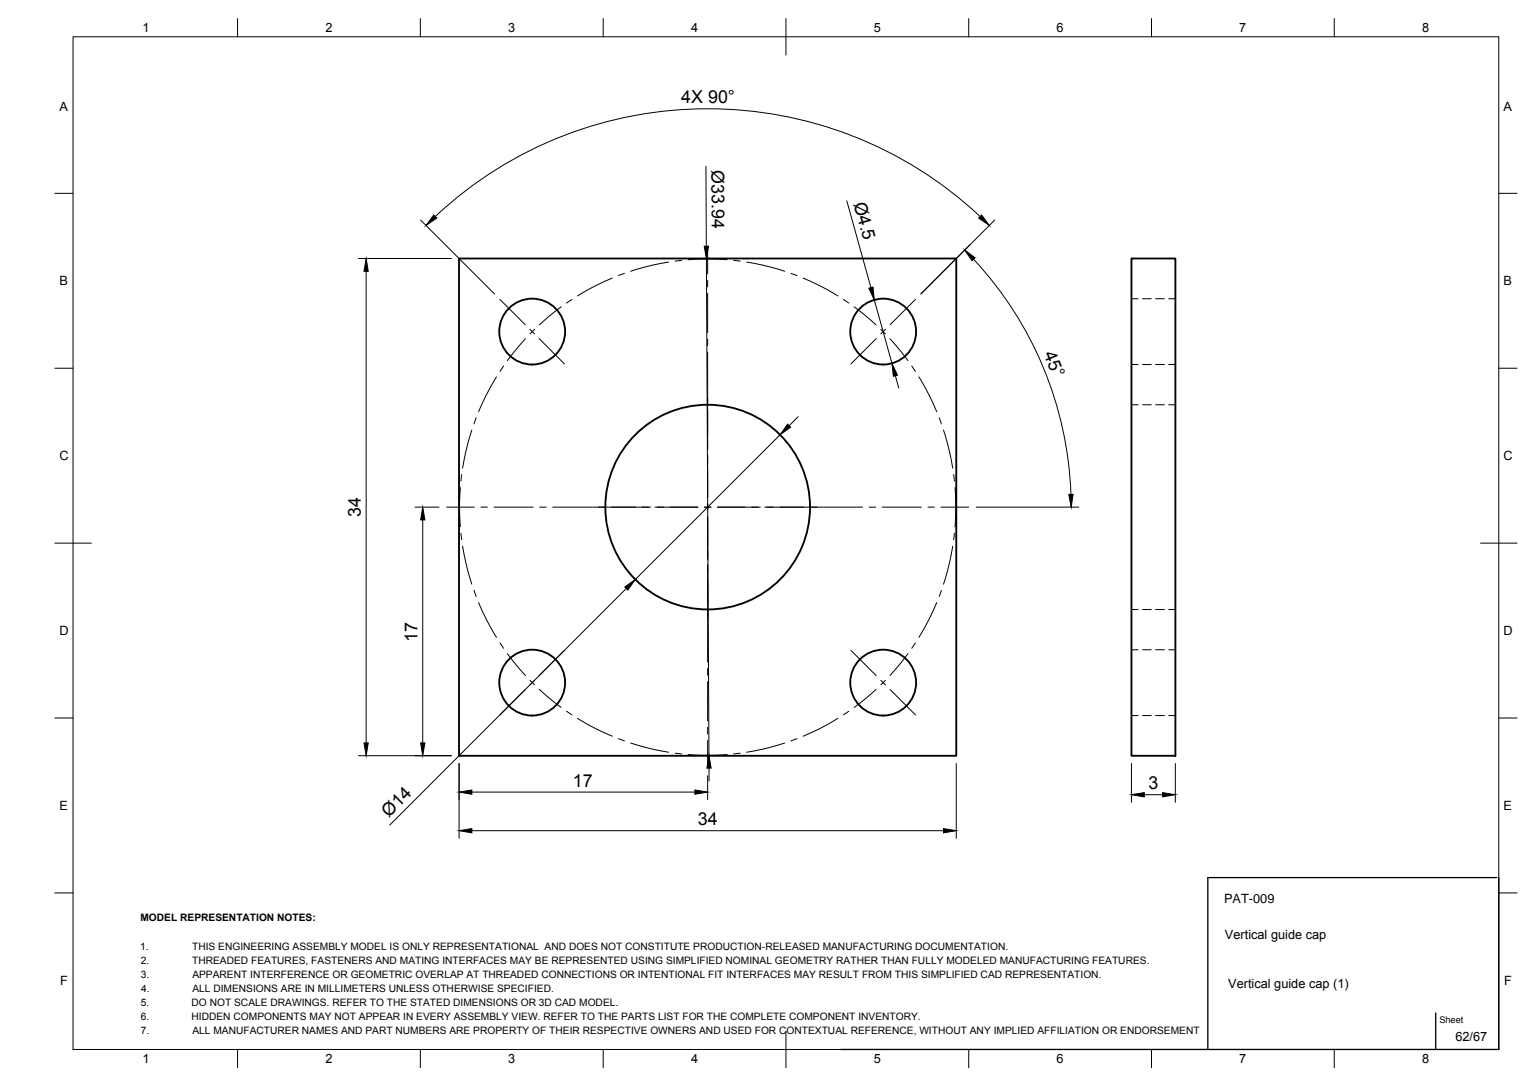
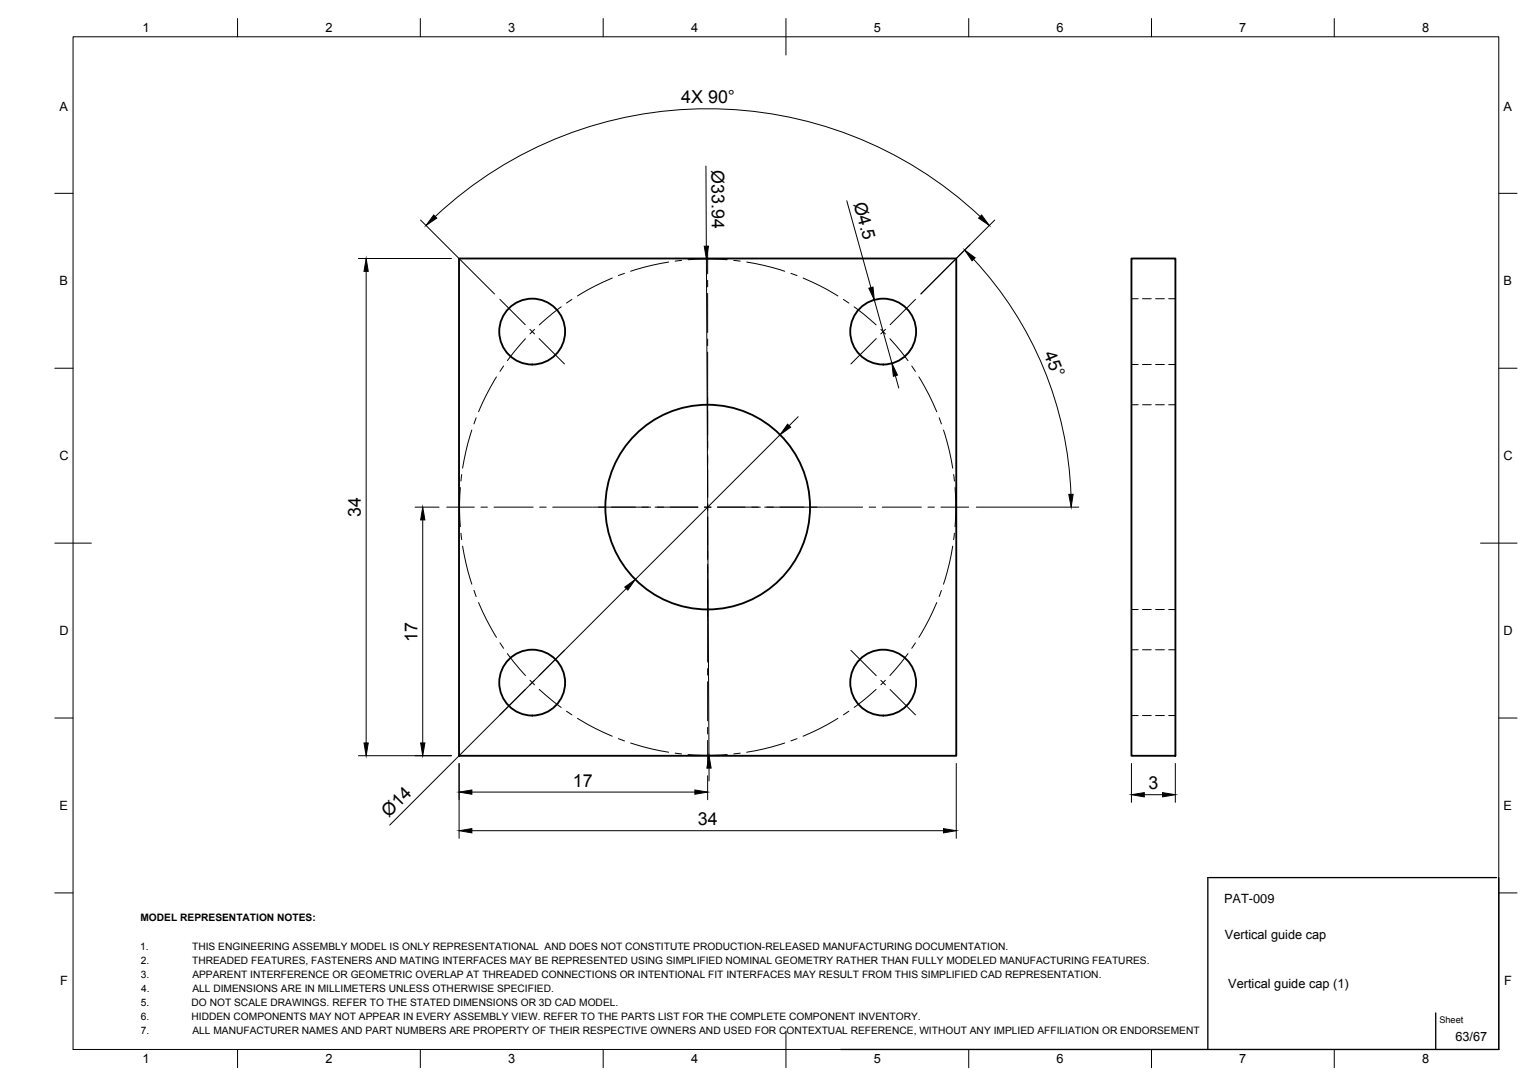
ISO-10303-21;
HEADER;
/* Generated by software containing ST-Developer
 * from STEP Tools, Inc. (www.steptools.com) 
 */

FILE_DESCRIPTION(
/* description */ ('Bell-crank linkage with push rods'),
/* implementation_level */ '2;1');

FILE_NAME(
/* name */ 'Vertical guide cap.step',
/* time_stamp */ '2026-10-28T03:25:15-07:00',
/* author */ (''),
/* organization */ (''),
/* preprocessor_version */ 'ST-DEVELOPER v20.2',
/* originating_system */ 'Autodesk Translation Framework v15.17.0.0',
/* authorisation */ '');

FILE_SCHEMA (('AUTOMOTIVE_DESIGN { 1 0 10303 214 3 1 1 }'));
ENDSEC;

DATA;
#10=MECHANICAL_DESIGN_GEOMETRIC_PRESENTATION_REPRESENTATION('',(#657),#16678);
#541=SHAPE_REPRESENTATION_RELATIONSHIP('SRR','None',#16963,#595);
#595=ADVANCED_BREP_SHAPE_REPRESENTATION('',(#717),#16668);
#657=STYLED_ITEM('',(#17277),#717);
#717=MANIFOLD_SOLID_BREP('Body1',#8849);
#925=FACE_BOUND('',#2413,.T.);
#926=FACE_BOUND('',#2414,.T.);
#927=FACE_BOUND('',#2415,.T.);
#928=FACE_BOUND('',#2416,.T.);
#929=FACE_BOUND('',#2417,.T.);
#930=FACE_BOUND('',#2420,.T.);
#931=FACE_BOUND('',#2421,.T.);
#932=FACE_BOUND('',#2422,.T.);
#933=FACE_BOUND('',#2423,.T.);
#934=FACE_BOUND('',#2424,.T.);
#1196=PLANE('',#10393);
#1197=PLANE('',#10394);
#1198=PLANE('',#10395);
#1199=PLANE('',#10396);
#1200=PLANE('',#10397);
#1201=PLANE('',#10398);
#1685=FACE_OUTER_BOUND('',#2407,.T.);
#1686=FACE_OUTER_BOUND('',#2408,.T.);
#1687=FACE_OUTER_BOUND('',#2409,.T.);
#1688=FACE_OUTER_BOUND('',#2410,.T.);
#1689=FACE_OUTER_BOUND('',#2411,.T.);
#1690=FACE_OUTER_BOUND('',#2412,.T.);
#1691=FACE_OUTER_BOUND('',#2418,.T.);
#1692=FACE_OUTER_BOUND('',#2419,.T.);
#1693=FACE_OUTER_BOUND('',#2425,.T.);
#1694=FACE_OUTER_BOUND('',#2426,.T.);
#1695=FACE_OUTER_BOUND('',#2427,.T.);
#2407=EDGE_LOOP('',(#7743,#7744,#7745,#7746));
#2408=EDGE_LOOP('',(#7747,#7748,#7749,#7750));
#2409=EDGE_LOOP('',(#7751,#7752,#7753,#7754));
#2410=EDGE_LOOP('',(#7755,#7756,#7757,#7758));
#2411=EDGE_LOOP('',(#7759,#7760,#7761,#7762));
#2412=EDGE_LOOP('',(#7763,#7764,#7765,#7766));
#2413=EDGE_LOOP('',(#7767));
#2414=EDGE_LOOP('',(#7768));
#2415=EDGE_LOOP('',(#7769));
#2416=EDGE_LOOP('',(#7770));
#2417=EDGE_LOOP('',(#7771));
#2418=EDGE_LOOP('',(#7772,#7773,#7774,#7775));
#2419=EDGE_LOOP('',(#7776,#7777,#7778,#7779));
#2420=EDGE_LOOP('',(#7780));
#2421=EDGE_LOOP('',(#7781));
#2422=EDGE_LOOP('',(#7782));
#2423=EDGE_LOOP('',(#7783));
#2424=EDGE_LOOP('',(#7784));
#2425=EDGE_LOOP('',(#7785,#7786,#7787,#7788));
#2426=EDGE_LOOP('',(#7789,#7790,#7791,#7792));
#2427=EDGE_LOOP('',(#7793,#7794,#7795,#7796));
#2988=LINE('',#16103,#3537);
#2989=LINE('',#16109,#3538);
#2990=LINE('',#16115,#3539);
#2991=LINE('',#16121,#3540);
#2992=LINE('',#16127,#3541);
#2993=LINE('',#16132,#3542);
#2994=LINE('',#16134,#3543);
#2995=LINE('',#16136,#3544);
#2996=LINE('',#16137,#3545);
#2997=LINE('',#16140,#3546);
#2998=LINE('',#16142,#3547);
#2999=LINE('',#16143,#3548);
#3000=LINE('',#16146,#3549);
#3001=LINE('',#16148,#3550);
#3002=LINE('',#16149,#3551);
#3003=LINE('',#16151,#3552);
#3004=LINE('',#16152,#3553);
#3537=VECTOR('',#12938,0.225);
#3538=VECTOR('',#12945,0.225);
#3539=VECTOR('',#12952,0.225);
#3540=VECTOR('',#12959,0.225);
#3541=VECTOR('',#12966,0.7);
#3542=VECTOR('',#12971,1.);
#3543=VECTOR('',#12972,1.);
#3544=VECTOR('',#12973,1.);
#3545=VECTOR('',#12974,1.);
#3546=VECTOR('',#12977,1.);
#3547=VECTOR('',#12978,1.);
#3548=VECTOR('',#12979,1.);
#3549=VECTOR('',#12982,1.);
#3550=VECTOR('',#12983,1.);
#3551=VECTOR('',#12984,1.);
#3552=VECTOR('',#12987,1.);
#3553=VECTOR('',#12988,1.);
#4051=CIRCLE('',#10379,0.225);
#4052=CIRCLE('',#10380,0.225);
#4053=CIRCLE('',#10382,0.225);
#4054=CIRCLE('',#10383,0.225);
#4055=CIRCLE('',#10385,0.225);
#4056=CIRCLE('',#10386,0.225);
#4057=CIRCLE('',#10388,0.225);
#4058=CIRCLE('',#10389,0.225);
#4059=CIRCLE('',#10391,0.7);
#4060=CIRCLE('',#10392,0.7);
#4726=VERTEX_POINT('',#16100);
#4727=VERTEX_POINT('',#16102);
#4728=VERTEX_POINT('',#16106);
#4729=VERTEX_POINT('',#16108);
#4730=VERTEX_POINT('',#16112);
#4731=VERTEX_POINT('',#16114);
#4732=VERTEX_POINT('',#16118);
#4733=VERTEX_POINT('',#16120);
#4734=VERTEX_POINT('',#16124);
#4735=VERTEX_POINT('',#16126);
#4736=VERTEX_POINT('',#16130);
#4737=VERTEX_POINT('',#16131);
#4738=VERTEX_POINT('',#16133);
#4739=VERTEX_POINT('',#16135);
#4740=VERTEX_POINT('',#16139);
#4741=VERTEX_POINT('',#16141);
#4742=VERTEX_POINT('',#16145);
#4743=VERTEX_POINT('',#16147);
#5749=EDGE_CURVE('',#4726,#4726,#4051,.T.);
#5750=EDGE_CURVE('',#4726,#4727,#2988,.T.);
#5751=EDGE_CURVE('',#4727,#4727,#4052,.T.);
#5752=EDGE_CURVE('',#4728,#4728,#4053,.T.);
#5753=EDGE_CURVE('',#4728,#4729,#2989,.T.);
#5754=EDGE_CURVE('',#4729,#4729,#4054,.T.);
#5755=EDGE_CURVE('',#4730,#4730,#4055,.T.);
#5756=EDGE_CURVE('',#4730,#4731,#2990,.T.);
#5757=EDGE_CURVE('',#4731,#4731,#4056,.T.);
#5758=EDGE_CURVE('',#4732,#4732,#4057,.T.);
#5759=EDGE_CURVE('',#4732,#4733,#2991,.T.);
#5760=EDGE_CURVE('',#4733,#4733,#4058,.T.);
#5761=EDGE_CURVE('',#4734,#4734,#4059,.T.);
#5762=EDGE_CURVE('',#4734,#4735,#2992,.T.);
#5763=EDGE_CURVE('',#4735,#4735,#4060,.T.);
#5764=EDGE_CURVE('',#4736,#4737,#2993,.T.);
#5765=EDGE_CURVE('',#4737,#4738,#2994,.T.);
#5766=EDGE_CURVE('',#4739,#4738,#2995,.T.);
#5767=EDGE_CURVE('',#4736,#4739,#2996,.T.);
#5768=EDGE_CURVE('',#4740,#4736,#2997,.T.);
#5769=EDGE_CURVE('',#4741,#4739,#2998,.T.);
#5770=EDGE_CURVE('',#4740,#4741,#2999,.T.);
#5771=EDGE_CURVE('',#4742,#4740,#3000,.T.);
#5772=EDGE_CURVE('',#4743,#4741,#3001,.T.);
#5773=EDGE_CURVE('',#4742,#4743,#3002,.T.);
#5774=EDGE_CURVE('',#4737,#4742,#3003,.T.);
#5775=EDGE_CURVE('',#4738,#4743,#3004,.T.);
#7743=ORIENTED_EDGE('',*,*,#5749,.F.);
#7744=ORIENTED_EDGE('',*,*,#5750,.T.);
#7745=ORIENTED_EDGE('',*,*,#5751,.F.);
#7746=ORIENTED_EDGE('',*,*,#5750,.F.);
#7747=ORIENTED_EDGE('',*,*,#5752,.F.);
#7748=ORIENTED_EDGE('',*,*,#5753,.T.);
#7749=ORIENTED_EDGE('',*,*,#5754,.F.);
#7750=ORIENTED_EDGE('',*,*,#5753,.F.);
#7751=ORIENTED_EDGE('',*,*,#5755,.F.);
#7752=ORIENTED_EDGE('',*,*,#5756,.T.);
#7753=ORIENTED_EDGE('',*,*,#5757,.F.);
#7754=ORIENTED_EDGE('',*,*,#5756,.F.);
#7755=ORIENTED_EDGE('',*,*,#5758,.F.);
#7756=ORIENTED_EDGE('',*,*,#5759,.T.);
#7757=ORIENTED_EDGE('',*,*,#5760,.F.);
#7758=ORIENTED_EDGE('',*,*,#5759,.F.);
#7759=ORIENTED_EDGE('',*,*,#5761,.F.);
#7760=ORIENTED_EDGE('',*,*,#5762,.T.);
#7761=ORIENTED_EDGE('',*,*,#5763,.F.);
#7762=ORIENTED_EDGE('',*,*,#5762,.F.);
#7763=ORIENTED_EDGE('',*,*,#5764,.T.);
#7764=ORIENTED_EDGE('',*,*,#5765,.T.);
#7765=ORIENTED_EDGE('',*,*,#5766,.F.);
#7766=ORIENTED_EDGE('',*,*,#5767,.F.);
#7767=ORIENTED_EDGE('',*,*,#5763,.T.);
#7768=ORIENTED_EDGE('',*,*,#5760,.T.);
#7769=ORIENTED_EDGE('',*,*,#5757,.T.);
#7770=ORIENTED_EDGE('',*,*,#5754,.T.);
#7771=ORIENTED_EDGE('',*,*,#5751,.T.);
#7772=ORIENTED_EDGE('',*,*,#5768,.T.);
#7773=ORIENTED_EDGE('',*,*,#5767,.T.);
#7774=ORIENTED_EDGE('',*,*,#5769,.F.);
#7775=ORIENTED_EDGE('',*,*,#5770,.F.);
#7776=ORIENTED_EDGE('',*,*,#5771,.T.);
#7777=ORIENTED_EDGE('',*,*,#5770,.T.);
#7778=ORIENTED_EDGE('',*,*,#5772,.F.);
#7779=ORIENTED_EDGE('',*,*,#5773,.F.);
#7780=ORIENTED_EDGE('',*,*,#5761,.T.);
#7781=ORIENTED_EDGE('',*,*,#5758,.T.);
#7782=ORIENTED_EDGE('',*,*,#5755,.T.);
#7783=ORIENTED_EDGE('',*,*,#5752,.T.);
#7784=ORIENTED_EDGE('',*,*,#5749,.T.);
#7785=ORIENTED_EDGE('',*,*,#5774,.T.);
#7786=ORIENTED_EDGE('',*,*,#5773,.T.);
#7787=ORIENTED_EDGE('',*,*,#5775,.F.);
#7788=ORIENTED_EDGE('',*,*,#5765,.F.);
#7789=ORIENTED_EDGE('',*,*,#5775,.T.);
#7790=ORIENTED_EDGE('',*,*,#5772,.T.);
#7791=ORIENTED_EDGE('',*,*,#5769,.T.);
#7792=ORIENTED_EDGE('',*,*,#5766,.T.);
#7793=ORIENTED_EDGE('',*,*,#5774,.F.);
#7794=ORIENTED_EDGE('',*,*,#5764,.F.);
#7795=ORIENTED_EDGE('',*,*,#5768,.F.);
#7796=ORIENTED_EDGE('',*,*,#5771,.F.);
#8242=CYLINDRICAL_SURFACE('',#10378,0.225);
#8243=CYLINDRICAL_SURFACE('',#10381,0.225);
#8244=CYLINDRICAL_SURFACE('',#10384,0.225);
#8245=CYLINDRICAL_SURFACE('',#10387,0.225);
#8246=CYLINDRICAL_SURFACE('',#10390,0.7);
#8710=ADVANCED_FACE('',(#1685),#8242,.F.);
#8711=ADVANCED_FACE('',(#1686),#8243,.F.);
#8712=ADVANCED_FACE('',(#1687),#8244,.F.);
#8713=ADVANCED_FACE('',(#1688),#8245,.F.);
#8714=ADVANCED_FACE('',(#1689),#8246,.F.);
#8715=ADVANCED_FACE('',(#1690,#925,#926,#927,#928,#929),#1196,.T.);
#8716=ADVANCED_FACE('',(#1691),#1197,.T.);
#8717=ADVANCED_FACE('',(#1692,#930,#931,#932,#933,#934),#1198,.T.);
#8718=ADVANCED_FACE('',(#1693),#1199,.T.);
#8719=ADVANCED_FACE('',(#1694),#1200,.T.);
#8720=ADVANCED_FACE('',(#1695),#1201,.F.);
#8849=CLOSED_SHELL('',(#8710,#8711,#8712,#8713,#8714,#8715,#8716,#8717,
#8718,#8719,#8720));
#10377=AXIS2_PLACEMENT_3D('',#16098,#12932,#12933);
#10378=AXIS2_PLACEMENT_3D('',#16099,#12934,#12935);
#10379=AXIS2_PLACEMENT_3D('',#16101,#12936,#12937);
#10380=AXIS2_PLACEMENT_3D('',#16104,#12939,#12940);
#10381=AXIS2_PLACEMENT_3D('',#16105,#12941,#12942);
#10382=AXIS2_PLACEMENT_3D('',#16107,#12943,#12944);
#10383=AXIS2_PLACEMENT_3D('',#16110,#12946,#12947);
#10384=AXIS2_PLACEMENT_3D('',#16111,#12948,#12949);
#10385=AXIS2_PLACEMENT_3D('',#16113,#12950,#12951);
#10386=AXIS2_PLACEMENT_3D('',#16116,#12953,#12954);
#10387=AXIS2_PLACEMENT_3D('',#16117,#12955,#12956);
#10388=AXIS2_PLACEMENT_3D('',#16119,#12957,#12958);
#10389=AXIS2_PLACEMENT_3D('',#16122,#12960,#12961);
#10390=AXIS2_PLACEMENT_3D('',#16123,#12962,#12963);
#10391=AXIS2_PLACEMENT_3D('',#16125,#12964,#12965);
#10392=AXIS2_PLACEMENT_3D('',#16128,#12967,#12968);
#10393=AXIS2_PLACEMENT_3D('',#16129,#12969,#12970);
#10394=AXIS2_PLACEMENT_3D('',#16138,#12975,#12976);
#10395=AXIS2_PLACEMENT_3D('',#16144,#12980,#12981);
#10396=AXIS2_PLACEMENT_3D('',#16150,#12985,#12986);
#10397=AXIS2_PLACEMENT_3D('',#16153,#12989,#12990);
#10398=AXIS2_PLACEMENT_3D('',#16154,#12991,#12992);
#12932=DIRECTION('axis',(0.,0.,1.));
#12933=DIRECTION('refdir',(1.,0.,0.));
#12934=DIRECTION('center_axis',(0.,1.,0.));
#12935=DIRECTION('ref_axis',(1.,0.,0.));
#12936=DIRECTION('center_axis',(0.,1.,0.));
#12937=DIRECTION('ref_axis',(1.,0.,0.));
#12938=DIRECTION('',(0.,1.,0.));
#12939=DIRECTION('center_axis',(0.,-1.,0.));
#12940=DIRECTION('ref_axis',(1.,0.,0.));
#12941=DIRECTION('center_axis',(0.,1.,0.));
#12942=DIRECTION('ref_axis',(1.,0.,0.));
#12943=DIRECTION('center_axis',(0.,1.,0.));
#12944=DIRECTION('ref_axis',(1.,0.,0.));
#12945=DIRECTION('',(0.,1.,0.));
#12946=DIRECTION('center_axis',(0.,-1.,0.));
#12947=DIRECTION('ref_axis',(1.,0.,0.));
#12948=DIRECTION('center_axis',(0.,1.,0.));
#12949=DIRECTION('ref_axis',(1.,0.,0.));
#12950=DIRECTION('center_axis',(0.,1.,0.));
#12951=DIRECTION('ref_axis',(1.,0.,0.));
#12952=DIRECTION('',(0.,1.,0.));
#12953=DIRECTION('center_axis',(0.,-1.,0.));
#12954=DIRECTION('ref_axis',(1.,0.,0.));
#12955=DIRECTION('center_axis',(0.,1.,0.));
#12956=DIRECTION('ref_axis',(1.,0.,0.));
#12957=DIRECTION('center_axis',(0.,1.,0.));
#12958=DIRECTION('ref_axis',(1.,0.,0.));
#12959=DIRECTION('',(0.,1.,0.));
#12960=DIRECTION('center_axis',(0.,-1.,0.));
#12961=DIRECTION('ref_axis',(1.,0.,0.));
#12962=DIRECTION('center_axis',(0.,1.,0.));
#12963=DIRECTION('ref_axis',(1.,0.,0.));
#12964=DIRECTION('center_axis',(0.,1.,0.));
#12965=DIRECTION('ref_axis',(1.,0.,0.));
#12966=DIRECTION('',(0.,1.,0.));
#12967=DIRECTION('center_axis',(0.,-1.,0.));
#12968=DIRECTION('ref_axis',(1.,0.,0.));
#12969=DIRECTION('center_axis',(0.,1.,0.));
#12970=DIRECTION('ref_axis',(-1.,0.,0.));
#12971=DIRECTION('',(-1.,0.,0.));
#12972=DIRECTION('',(0.,0.,1.));
#12973=DIRECTION('',(-1.,0.,0.));
#12974=DIRECTION('',(0.,0.,1.));
#12975=DIRECTION('center_axis',(1.,0.,0.));
#12976=DIRECTION('ref_axis',(0.,1.,0.));
#12977=DIRECTION('',(0.,1.,0.));
#12978=DIRECTION('',(0.,1.,0.));
#12979=DIRECTION('',(0.,0.,1.));
#12980=DIRECTION('center_axis',(0.,-1.,0.));
#12981=DIRECTION('ref_axis',(1.,0.,0.));
#12982=DIRECTION('',(1.,0.,0.));
#12983=DIRECTION('',(1.,0.,0.));
#12984=DIRECTION('',(0.,0.,1.));
#12985=DIRECTION('center_axis',(-1.,0.,0.));
#12986=DIRECTION('ref_axis',(0.,-1.,0.));
#12987=DIRECTION('',(0.,-1.,0.));
#12988=DIRECTION('',(0.,-1.,0.));
#12989=DIRECTION('center_axis',(0.,0.,1.));
#12990=DIRECTION('ref_axis',(1.,0.,0.));
#12991=DIRECTION('center_axis',(0.,0.,1.));
#12992=DIRECTION('ref_axis',(1.,0.,0.));
#16098=CARTESIAN_POINT('',(0.,0.,0.));
#16099=CARTESIAN_POINT('Origin',(5.2,10.1,2.8));
#16100=CARTESIAN_POINT('',(4.975,10.2,2.8));
#16101=CARTESIAN_POINT('Origin',(5.2,10.2,2.8));
#16102=CARTESIAN_POINT('',(4.975,10.5,2.8));
#16103=CARTESIAN_POINT('',(4.975,10.1,2.8));
#16104=CARTESIAN_POINT('Origin',(5.2,10.5,2.8));
#16105=CARTESIAN_POINT('Origin',(2.8,10.1,5.2));
#16106=CARTESIAN_POINT('',(2.575,10.2,5.2));
#16107=CARTESIAN_POINT('Origin',(2.8,10.2,5.2));
#16108=CARTESIAN_POINT('',(2.575,10.5,5.2));
#16109=CARTESIAN_POINT('',(2.575,10.1,5.2));
#16110=CARTESIAN_POINT('Origin',(2.8,10.5,5.2));
#16111=CARTESIAN_POINT('Origin',(2.8,10.1,2.8));
#16112=CARTESIAN_POINT('',(2.575,10.2,2.8));
#16113=CARTESIAN_POINT('Origin',(2.8,10.2,2.8));
#16114=CARTESIAN_POINT('',(2.575,10.5,2.8));
#16115=CARTESIAN_POINT('',(2.575,10.1,2.8));
#16116=CARTESIAN_POINT('Origin',(2.8,10.5,2.8));
#16117=CARTESIAN_POINT('Origin',(5.2,10.1,5.2));
#16118=CARTESIAN_POINT('',(4.975,10.2,5.2));
#16119=CARTESIAN_POINT('Origin',(5.2,10.2,5.2));
#16120=CARTESIAN_POINT('',(4.975,10.5,5.2));
#16121=CARTESIAN_POINT('',(4.975,10.1,5.2));
#16122=CARTESIAN_POINT('Origin',(5.2,10.5,5.2));
#16123=CARTESIAN_POINT('Origin',(4.,10.1,4.));
#16124=CARTESIAN_POINT('',(3.3,10.2,4.));
#16125=CARTESIAN_POINT('Origin',(4.,10.2,4.));
#16126=CARTESIAN_POINT('',(3.3,10.5,4.));
#16127=CARTESIAN_POINT('',(3.3,10.1,4.));
#16128=CARTESIAN_POINT('Origin',(4.,10.5,4.));
#16129=CARTESIAN_POINT('Origin',(5.7,10.5,2.3));
#16130=CARTESIAN_POINT('',(5.7,10.5,2.3));
#16131=CARTESIAN_POINT('',(2.3,10.5,2.3));
#16132=CARTESIAN_POINT('',(5.7,10.5,2.3));
#16133=CARTESIAN_POINT('',(2.3,10.5,5.7));
#16134=CARTESIAN_POINT('',(2.3,10.5,2.3));
#16135=CARTESIAN_POINT('',(5.7,10.5,5.7));
#16136=CARTESIAN_POINT('',(5.7,10.5,5.7));
#16137=CARTESIAN_POINT('',(5.7,10.5,2.3));
#16138=CARTESIAN_POINT('Origin',(5.7,10.2,2.3));
#16139=CARTESIAN_POINT('',(5.7,10.2,2.3));
#16140=CARTESIAN_POINT('',(5.7,10.2,2.3));
#16141=CARTESIAN_POINT('',(5.7,10.2,5.7));
#16142=CARTESIAN_POINT('',(5.7,10.2,5.7));
#16143=CARTESIAN_POINT('',(5.7,10.2,2.3));
#16144=CARTESIAN_POINT('Origin',(2.3,10.2,2.3));
#16145=CARTESIAN_POINT('',(2.3,10.2,2.3));
#16146=CARTESIAN_POINT('',(2.3,10.2,2.3));
#16147=CARTESIAN_POINT('',(2.3,10.2,5.7));
#16148=CARTESIAN_POINT('',(2.3,10.2,5.7));
#16149=CARTESIAN_POINT('',(2.3,10.2,2.3));
#16150=CARTESIAN_POINT('Origin',(2.3,10.5,2.3));
#16151=CARTESIAN_POINT('',(2.3,10.5,2.3));
#16152=CARTESIAN_POINT('',(2.3,10.5,5.7));
#16153=CARTESIAN_POINT('Origin',(4.,10.35,5.7));
#16154=CARTESIAN_POINT('Origin',(4.,10.35,2.3));
#16604=UNCERTAINTY_MEASURE_WITH_UNIT(LENGTH_MEASURE(0.001),#16679,
'DISTANCE_ACCURACY_VALUE',
'Maximum model space distance between geometric entities at asserted c
onnectivities');
#16614=UNCERTAINTY_MEASURE_WITH_UNIT(LENGTH_MEASURE(0.001),#16679,
'DISTANCE_ACCURACY_VALUE',
'Maximum model space distance between geometric entities at asserted c
onnectivities');
#16668=(
GEOMETRIC_REPRESENTATION_CONTEXT(3)
GLOBAL_UNCERTAINTY_ASSIGNED_CONTEXT((#16604))
GLOBAL_UNIT_ASSIGNED_CONTEXT((#16679,#16681,#16682))
REPRESENTATION_CONTEXT('','3D')
);
#16678=(
GEOMETRIC_REPRESENTATION_CONTEXT(3)
GLOBAL_UNCERTAINTY_ASSIGNED_CONTEXT((#16614))
GLOBAL_UNIT_ASSIGNED_CONTEXT((#16679,#16681,#16682))
REPRESENTATION_CONTEXT('','3D')
);
#16679=(
LENGTH_UNIT()
NAMED_UNIT(*)
SI_UNIT(.CENTI.,.METRE.)
);
#16681=(
NAMED_UNIT(*)
PLANE_ANGLE_UNIT()
SI_UNIT($,.RADIAN.)
);
#16682=(
NAMED_UNIT(*)
SI_UNIT($,.STERADIAN.)
SOLID_ANGLE_UNIT()
);
#16736=SHAPE_DEFINITION_REPRESENTATION(#16810,#16963);
#16810=PRODUCT_DEFINITION_SHAPE('',$,#17027);
#16963=SHAPE_REPRESENTATION('',(#10377),#16668);
#16973=PRODUCT_DEFINITION_CONTEXT('part definition',#17164,'design');
#17027=PRODUCT_DEFINITION('Vertical guide cap','Vertical guide cap',#17090,
#16973);
#17090=PRODUCT_DEFINITION_FORMATION('',$,#17219);
#17164=APPLICATION_CONTEXT(
'Core Data for Automotive Mechanical Design Process');
#17165=PRODUCT_CONTEXT('part definition',#17164,'mechanical');
#17219=PRODUCT('Vertical guide cap','Vertical guide cap',
'Vertical guide cap',(#17165));
#17271=COLOUR_RGB('Light Blue',0.38,0.62,0.78);
#17272=FILL_AREA_STYLE_COLOUR('',#17271);
#17273=FILL_AREA_STYLE('',(#17272));
#17274=SURFACE_STYLE_FILL_AREA(#17273);
#17275=SURFACE_SIDE_STYLE('',(#17274));
#17276=SURFACE_STYLE_USAGE(.BOTH.,#17275);
#17277=PRESENTATION_STYLE_ASSIGNMENT((#17276));
ENDSEC;
END-ISO-10303-21;
